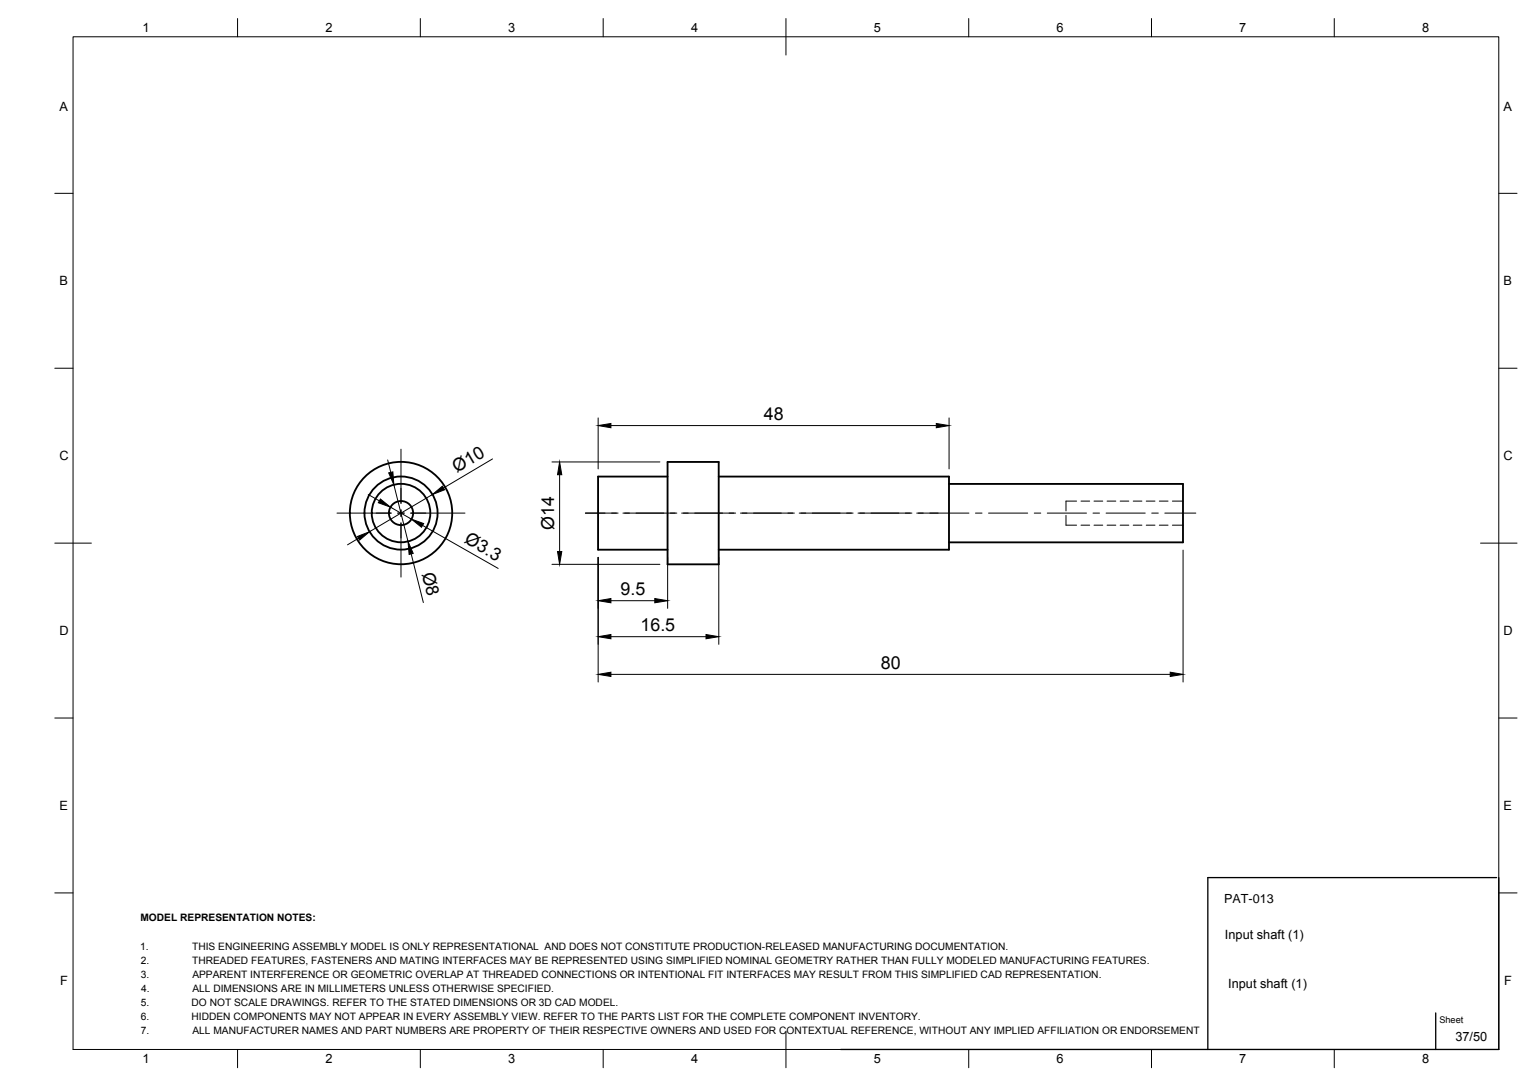
ISO-10303-21;
HEADER;
/* Generated by software containing ST-Developer
 * from STEP Tools, Inc. (www.steptools.com) 
 */

FILE_DESCRIPTION(
/* description */ ('Belt-driven linear axis on 2020 extrusion'),
/* implementation_level */ '2;1');

FILE_NAME(
/* name */ 'Input shaft (1).step',
/* time_stamp */ '2026-10-28T03:26:09-07:00',
/* author */ (''),
/* organization */ (''),
/* preprocessor_version */ 'ST-DEVELOPER v20.2',
/* originating_system */ 'Autodesk Translation Framework v15.17.0.0',
/* authorisation */ '');

FILE_SCHEMA (('AUTOMOTIVE_DESIGN { 1 0 10303 214 3 1 1 }'));
ENDSEC;

DATA;
#10=MECHANICAL_DESIGN_GEOMETRIC_PRESENTATION_REPRESENTATION('',(#649),#20096);
#547=SHAPE_REPRESENTATION_RELATIONSHIP('SRR','None',#20346,#593);
#593=ADVANCED_BREP_SHAPE_REPRESENTATION('',(#704),#20077);
#649=STYLED_ITEM('',(#20650),#704);
#704=MANIFOLD_SOLID_BREP('Body1',#10963);
#840=FACE_BOUND('',#2396,.T.);
#841=FACE_BOUND('',#2398,.T.);
#842=FACE_BOUND('',#2403,.T.);
#843=FACE_BOUND('',#2407,.T.);
#1127=PLANE('',#12259);
#1128=PLANE('',#12260);
#1129=PLANE('',#12263);
#1130=PLANE('',#12272);
#1131=PLANE('',#12275);
#1132=PLANE('',#12276);
#1649=FACE_OUTER_BOUND('',#2393,.T.);
#1650=FACE_OUTER_BOUND('',#2394,.T.);
#1651=FACE_OUTER_BOUND('',#2395,.T.);
#1652=FACE_OUTER_BOUND('',#2397,.T.);
#1653=FACE_OUTER_BOUND('',#2399,.T.);
#1654=FACE_OUTER_BOUND('',#2400,.T.);
#1655=FACE_OUTER_BOUND('',#2401,.T.);
#1656=FACE_OUTER_BOUND('',#2402,.T.);
#1657=FACE_OUTER_BOUND('',#2404,.T.);
#1658=FACE_OUTER_BOUND('',#2405,.T.);
#1659=FACE_OUTER_BOUND('',#2406,.T.);
#2393=EDGE_LOOP('',(#9049,#9050,#9051,#9052));
#2394=EDGE_LOOP('',(#9053));
#2395=EDGE_LOOP('',(#9054));
#2396=EDGE_LOOP('',(#9055));
#2397=EDGE_LOOP('',(#9056));
#2398=EDGE_LOOP('',(#9057));
#2399=EDGE_LOOP('',(#9058,#9059,#9060,#9061));
#2400=EDGE_LOOP('',(#9062,#9063,#9064,#9065));
#2401=EDGE_LOOP('',(#9066,#9067,#9068,#9069));
#2402=EDGE_LOOP('',(#9070));
#2403=EDGE_LOOP('',(#9071));
#2404=EDGE_LOOP('',(#9072,#9073,#9074,#9075));
#2405=EDGE_LOOP('',(#9076));
#2406=EDGE_LOOP('',(#9077));
#2407=EDGE_LOOP('',(#9078));
#3218=LINE('',#18518,#4075);
#3219=LINE('',#18532,#4076);
#3220=LINE('',#18535,#4077);
#3221=LINE('',#18541,#4078);
#3222=LINE('',#18547,#4079);
#4075=VECTOR('',#14874,0.164999999999999);
#4076=VECTOR('',#14893,0.700000000000003);
#4077=VECTOR('',#14896,0.5);
#4078=VECTOR('',#14903,0.399999999999999);
#4079=VECTOR('',#14912,0.5);
#4704=CIRCLE('',#12257,0.164999999999999);
#4705=CIRCLE('',#12258,0.164999999999999);
#4706=CIRCLE('',#12261,0.700000000000003);
#4707=CIRCLE('',#12262,0.5);
#4708=CIRCLE('',#12264,0.700000000000003);
#4709=CIRCLE('',#12265,0.5);
#4710=CIRCLE('',#12268,0.5);
#4711=CIRCLE('',#12270,0.399999999999999);
#4712=CIRCLE('',#12271,0.399999999999999);
#4713=CIRCLE('',#12274,0.5);
#5499=VERTEX_POINT('',#18515);
#5500=VERTEX_POINT('',#18517);
#5501=VERTEX_POINT('',#18522);
#5502=VERTEX_POINT('',#18524);
#5503=VERTEX_POINT('',#18527);
#5504=VERTEX_POINT('',#18529);
#5505=VERTEX_POINT('',#18534);
#5506=VERTEX_POINT('',#18538);
#5507=VERTEX_POINT('',#18540);
#5508=VERTEX_POINT('',#18545);
#6739=EDGE_CURVE('',#5499,#5499,#4704,.T.);
#6740=EDGE_CURVE('',#5499,#5500,#3218,.T.);
#6741=EDGE_CURVE('',#5500,#5500,#4705,.T.);
#6742=EDGE_CURVE('',#5501,#5501,#4706,.T.);
#6743=EDGE_CURVE('',#5502,#5502,#4707,.T.);
#6744=EDGE_CURVE('',#5503,#5503,#4708,.T.);
#6745=EDGE_CURVE('',#5504,#5504,#4709,.T.);
#6746=EDGE_CURVE('',#5501,#5503,#3219,.T.);
#6747=EDGE_CURVE('',#5504,#5505,#3220,.T.);
#6748=EDGE_CURVE('',#5505,#5505,#4710,.T.);
#6749=EDGE_CURVE('',#5506,#5506,#4711,.T.);
#6750=EDGE_CURVE('',#5506,#5507,#3221,.T.);
#6751=EDGE_CURVE('',#5507,#5507,#4712,.T.);
#6752=EDGE_CURVE('',#5508,#5508,#4713,.T.);
#6753=EDGE_CURVE('',#5508,#5502,#3222,.T.);
#9049=ORIENTED_EDGE('',*,*,#6739,.F.);
#9050=ORIENTED_EDGE('',*,*,#6740,.T.);
#9051=ORIENTED_EDGE('',*,*,#6741,.T.);
#9052=ORIENTED_EDGE('',*,*,#6740,.F.);
#9053=ORIENTED_EDGE('',*,*,#6741,.F.);
#9054=ORIENTED_EDGE('',*,*,#6742,.T.);
#9055=ORIENTED_EDGE('',*,*,#6743,.F.);
#9056=ORIENTED_EDGE('',*,*,#6744,.F.);
#9057=ORIENTED_EDGE('',*,*,#6745,.F.);
#9058=ORIENTED_EDGE('',*,*,#6742,.F.);
#9059=ORIENTED_EDGE('',*,*,#6746,.T.);
#9060=ORIENTED_EDGE('',*,*,#6744,.T.);
#9061=ORIENTED_EDGE('',*,*,#6746,.F.);
#9062=ORIENTED_EDGE('',*,*,#6745,.T.);
#9063=ORIENTED_EDGE('',*,*,#6747,.T.);
#9064=ORIENTED_EDGE('',*,*,#6748,.T.);
#9065=ORIENTED_EDGE('',*,*,#6747,.F.);
#9066=ORIENTED_EDGE('',*,*,#6749,.F.);
#9067=ORIENTED_EDGE('',*,*,#6750,.T.);
#9068=ORIENTED_EDGE('',*,*,#6751,.T.);
#9069=ORIENTED_EDGE('',*,*,#6750,.F.);
#9070=ORIENTED_EDGE('',*,*,#6751,.F.);
#9071=ORIENTED_EDGE('',*,*,#6739,.T.);
#9072=ORIENTED_EDGE('',*,*,#6752,.F.);
#9073=ORIENTED_EDGE('',*,*,#6753,.T.);
#9074=ORIENTED_EDGE('',*,*,#6743,.T.);
#9075=ORIENTED_EDGE('',*,*,#6753,.F.);
#9076=ORIENTED_EDGE('',*,*,#6752,.T.);
#9077=ORIENTED_EDGE('',*,*,#6748,.F.);
#9078=ORIENTED_EDGE('',*,*,#6749,.T.);
#10213=CYLINDRICAL_SURFACE('',#12256,0.164999999999999);
#10214=CYLINDRICAL_SURFACE('',#12266,0.700000000000003);
#10215=CYLINDRICAL_SURFACE('',#12267,0.5);
#10216=CYLINDRICAL_SURFACE('',#12269,0.399999999999999);
#10217=CYLINDRICAL_SURFACE('',#12273,0.5);
#10700=ADVANCED_FACE('',(#1649),#10213,.F.);
#10701=ADVANCED_FACE('',(#1650),#1127,.F.);
#10702=ADVANCED_FACE('',(#1651,#840),#1128,.T.);
#10703=ADVANCED_FACE('',(#1652,#841),#1129,.F.);
#10704=ADVANCED_FACE('',(#1653),#10214,.T.);
#10705=ADVANCED_FACE('',(#1654),#10215,.T.);
#10706=ADVANCED_FACE('',(#1655),#10216,.T.);
#10707=ADVANCED_FACE('',(#1656,#842),#1130,.F.);
#10708=ADVANCED_FACE('',(#1657),#10217,.T.);
#10709=ADVANCED_FACE('',(#1658),#1131,.T.);
#10710=ADVANCED_FACE('',(#1659,#843),#1132,.F.);
#10963=CLOSED_SHELL('',(#10700,#10701,#10702,#10703,#10704,#10705,#10706,
#10707,#10708,#10709,#10710));
#12255=AXIS2_PLACEMENT_3D('',#18513,#14868,#14869);
#12256=AXIS2_PLACEMENT_3D('',#18514,#14870,#14871);
#12257=AXIS2_PLACEMENT_3D('',#18516,#14872,#14873);
#12258=AXIS2_PLACEMENT_3D('',#18519,#14875,#14876);
#12259=AXIS2_PLACEMENT_3D('',#18520,#14877,#14878);
#12260=AXIS2_PLACEMENT_3D('',#18521,#14879,#14880);
#12261=AXIS2_PLACEMENT_3D('',#18523,#14881,#14882);
#12262=AXIS2_PLACEMENT_3D('',#18525,#14883,#14884);
#12263=AXIS2_PLACEMENT_3D('',#18526,#14885,#14886);
#12264=AXIS2_PLACEMENT_3D('',#18528,#14887,#14888);
#12265=AXIS2_PLACEMENT_3D('',#18530,#14889,#14890);
#12266=AXIS2_PLACEMENT_3D('',#18531,#14891,#14892);
#12267=AXIS2_PLACEMENT_3D('',#18533,#14894,#14895);
#12268=AXIS2_PLACEMENT_3D('',#18536,#14897,#14898);
#12269=AXIS2_PLACEMENT_3D('',#18537,#14899,#14900);
#12270=AXIS2_PLACEMENT_3D('',#18539,#14901,#14902);
#12271=AXIS2_PLACEMENT_3D('',#18542,#14904,#14905);
#12272=AXIS2_PLACEMENT_3D('',#18543,#14906,#14907);
#12273=AXIS2_PLACEMENT_3D('',#18544,#14908,#14909);
#12274=AXIS2_PLACEMENT_3D('',#18546,#14910,#14911);
#12275=AXIS2_PLACEMENT_3D('',#18548,#14913,#14914);
#12276=AXIS2_PLACEMENT_3D('',#18549,#14915,#14916);
#14868=DIRECTION('axis',(0.,0.,1.));
#14869=DIRECTION('refdir',(1.,0.,0.));
#14870=DIRECTION('center_axis',(0.,1.,0.));
#14871=DIRECTION('ref_axis',(1.,0.,0.));
#14872=DIRECTION('center_axis',(0.,1.,0.));
#14873=DIRECTION('ref_axis',(1.,0.,0.));
#14874=DIRECTION('',(0.,1.,0.));
#14875=DIRECTION('center_axis',(0.,1.,0.));
#14876=DIRECTION('ref_axis',(1.,0.,0.));
#14877=DIRECTION('center_axis',(0.,1.,0.));
#14878=DIRECTION('ref_axis',(1.,0.,0.));
#14879=DIRECTION('center_axis',(0.,1.,0.));
#14880=DIRECTION('ref_axis',(1.,0.,0.));
#14881=DIRECTION('center_axis',(0.,1.,0.));
#14882=DIRECTION('ref_axis',(1.,0.,0.));
#14883=DIRECTION('center_axis',(0.,1.,0.));
#14884=DIRECTION('ref_axis',(1.,0.,0.));
#14885=DIRECTION('center_axis',(0.,1.,0.));
#14886=DIRECTION('ref_axis',(1.,0.,0.));
#14887=DIRECTION('center_axis',(0.,1.,0.));
#14888=DIRECTION('ref_axis',(1.,0.,0.));
#14889=DIRECTION('center_axis',(0.,-1.,0.));
#14890=DIRECTION('ref_axis',(1.,0.,0.));
#14891=DIRECTION('center_axis',(0.,1.,0.));
#14892=DIRECTION('ref_axis',(1.,0.,0.));
#14893=DIRECTION('',(0.,-1.,0.));
#14894=DIRECTION('center_axis',(0.,1.,0.));
#14895=DIRECTION('ref_axis',(1.,0.,0.));
#14896=DIRECTION('',(0.,-1.,0.));
#14897=DIRECTION('center_axis',(0.,1.,0.));
#14898=DIRECTION('ref_axis',(1.,0.,0.));
#14899=DIRECTION('center_axis',(0.,1.,0.));
#14900=DIRECTION('ref_axis',(1.,0.,0.));
#14901=DIRECTION('center_axis',(0.,1.,0.));
#14902=DIRECTION('ref_axis',(1.,0.,0.));
#14903=DIRECTION('',(0.,-1.,0.));
#14904=DIRECTION('center_axis',(0.,1.,0.));
#14905=DIRECTION('ref_axis',(1.,0.,0.));
#14906=DIRECTION('center_axis',(0.,1.,0.));
#14907=DIRECTION('ref_axis',(1.,0.,0.));
#14908=DIRECTION('center_axis',(0.,1.,0.));
#14909=DIRECTION('ref_axis',(1.,0.,0.));
#14910=DIRECTION('center_axis',(0.,1.,0.));
#14911=DIRECTION('ref_axis',(1.,0.,0.));
#14912=DIRECTION('',(0.,-1.,0.));
#14913=DIRECTION('center_axis',(0.,1.,0.));
#14914=DIRECTION('ref_axis',(1.,0.,0.));
#14915=DIRECTION('center_axis',(0.,1.,0.));
#14916=DIRECTION('ref_axis',(1.,0.,0.));
#18513=CARTESIAN_POINT('',(0.,0.,0.));
#18514=CARTESIAN_POINT('Origin',(32.,-5.1,7.));
#18515=CARTESIAN_POINT('',(31.835,-5.,7.));
#18516=CARTESIAN_POINT('Origin',(32.,-5.,7.));
#18517=CARTESIAN_POINT('',(31.835,-3.4,7.));
#18518=CARTESIAN_POINT('',(31.835,-5.1,7.));
#18519=CARTESIAN_POINT('Origin',(32.,-3.4,7.));
#18520=CARTESIAN_POINT('Origin',(32.,-3.4,7.));
#18521=CARTESIAN_POINT('Origin',(32.,2.05,7.));
#18522=CARTESIAN_POINT('',(31.3,2.05,7.));
#18523=CARTESIAN_POINT('Origin',(32.,2.05,7.));
#18524=CARTESIAN_POINT('',(31.5,2.05,7.));
#18525=CARTESIAN_POINT('Origin',(32.,2.05,7.));
#18526=CARTESIAN_POINT('Origin',(32.,1.35,7.));
#18527=CARTESIAN_POINT('',(31.3,1.35,7.));
#18528=CARTESIAN_POINT('Origin',(32.,1.35,7.));
#18529=CARTESIAN_POINT('',(31.5,1.35,7.));
#18530=CARTESIAN_POINT('Origin',(32.,1.35,7.));
#18531=CARTESIAN_POINT('Origin',(32.,1.35,7.));
#18532=CARTESIAN_POINT('',(31.3,1.35,7.));
#18533=CARTESIAN_POINT('Origin',(32.,-1.8,7.));
#18534=CARTESIAN_POINT('',(31.5,-1.8,7.));
#18535=CARTESIAN_POINT('',(31.5,-1.8,7.));
#18536=CARTESIAN_POINT('Origin',(32.,-1.8,7.));
#18537=CARTESIAN_POINT('Origin',(32.,-5.,7.));
#18538=CARTESIAN_POINT('',(31.6,-1.8,7.));
#18539=CARTESIAN_POINT('Origin',(32.,-1.8,7.));
#18540=CARTESIAN_POINT('',(31.6,-5.,7.));
#18541=CARTESIAN_POINT('',(31.6,-5.,7.));
#18542=CARTESIAN_POINT('Origin',(32.,-5.,7.));
#18543=CARTESIAN_POINT('Origin',(32.,-5.,7.));
#18544=CARTESIAN_POINT('Origin',(32.,-1.8,7.));
#18545=CARTESIAN_POINT('',(31.5,3.,7.));
#18546=CARTESIAN_POINT('Origin',(32.,3.,7.));
#18547=CARTESIAN_POINT('',(31.5,-1.8,7.));
#18548=CARTESIAN_POINT('Origin',(32.,3.,7.));
#18549=CARTESIAN_POINT('Origin',(32.,-1.8,7.));
#20023=UNCERTAINTY_MEASURE_WITH_UNIT(LENGTH_MEASURE(0.001),#20097,
'DISTANCE_ACCURACY_VALUE',
'Maximum model space distance between geometric entities at asserted c
onnectivities');
#20042=UNCERTAINTY_MEASURE_WITH_UNIT(LENGTH_MEASURE(0.001),#20097,
'DISTANCE_ACCURACY_VALUE',
'Maximum model space distance between geometric entities at asserted c
onnectivities');
#20077=(
GEOMETRIC_REPRESENTATION_CONTEXT(3)
GLOBAL_UNCERTAINTY_ASSIGNED_CONTEXT((#20023))
GLOBAL_UNIT_ASSIGNED_CONTEXT((#20097,#20099,#20100))
REPRESENTATION_CONTEXT('','3D')
);
#20096=(
GEOMETRIC_REPRESENTATION_CONTEXT(3)
GLOBAL_UNCERTAINTY_ASSIGNED_CONTEXT((#20042))
GLOBAL_UNIT_ASSIGNED_CONTEXT((#20097,#20099,#20100))
REPRESENTATION_CONTEXT('','3D')
);
#20097=(
LENGTH_UNIT()
NAMED_UNIT(*)
SI_UNIT(.CENTI.,.METRE.)
);
#20099=(
NAMED_UNIT(*)
PLANE_ANGLE_UNIT()
SI_UNIT($,.RADIAN.)
);
#20100=(
NAMED_UNIT(*)
SI_UNIT($,.STERADIAN.)
SOLID_ANGLE_UNIT()
);
#20135=SHAPE_DEFINITION_REPRESENTATION(#20193,#20346);
#20193=PRODUCT_DEFINITION_SHAPE('',$,#20400);
#20346=SHAPE_REPRESENTATION('',(#12255),#20077);
#20365=PRODUCT_DEFINITION_CONTEXT('part definition',#20526,'design');
#20400=PRODUCT_DEFINITION('Input shaft (1)','Input shaft (1)',#20453,#20365);
#20453=PRODUCT_DEFINITION_FORMATION('',$,#20562);
#20526=APPLICATION_CONTEXT(
'Core Data for Automotive Mechanical Design Process');
#20527=PRODUCT_CONTEXT('part definition',#20526,'mechanical');
#20562=PRODUCT('Input shaft (1)','Input shaft (1)','Input shaft (1)',(#20527));
#20644=COLOUR_RGB('Grey',0.48,0.52,0.57);
#20645=FILL_AREA_STYLE_COLOUR('',#20644);
#20646=FILL_AREA_STYLE('',(#20645));
#20647=SURFACE_STYLE_FILL_AREA(#20646);
#20648=SURFACE_SIDE_STYLE('',(#20647));
#20649=SURFACE_STYLE_USAGE(.BOTH.,#20648);
#20650=PRESENTATION_STYLE_ASSIGNMENT((#20649));
ENDSEC;
END-ISO-10303-21;
